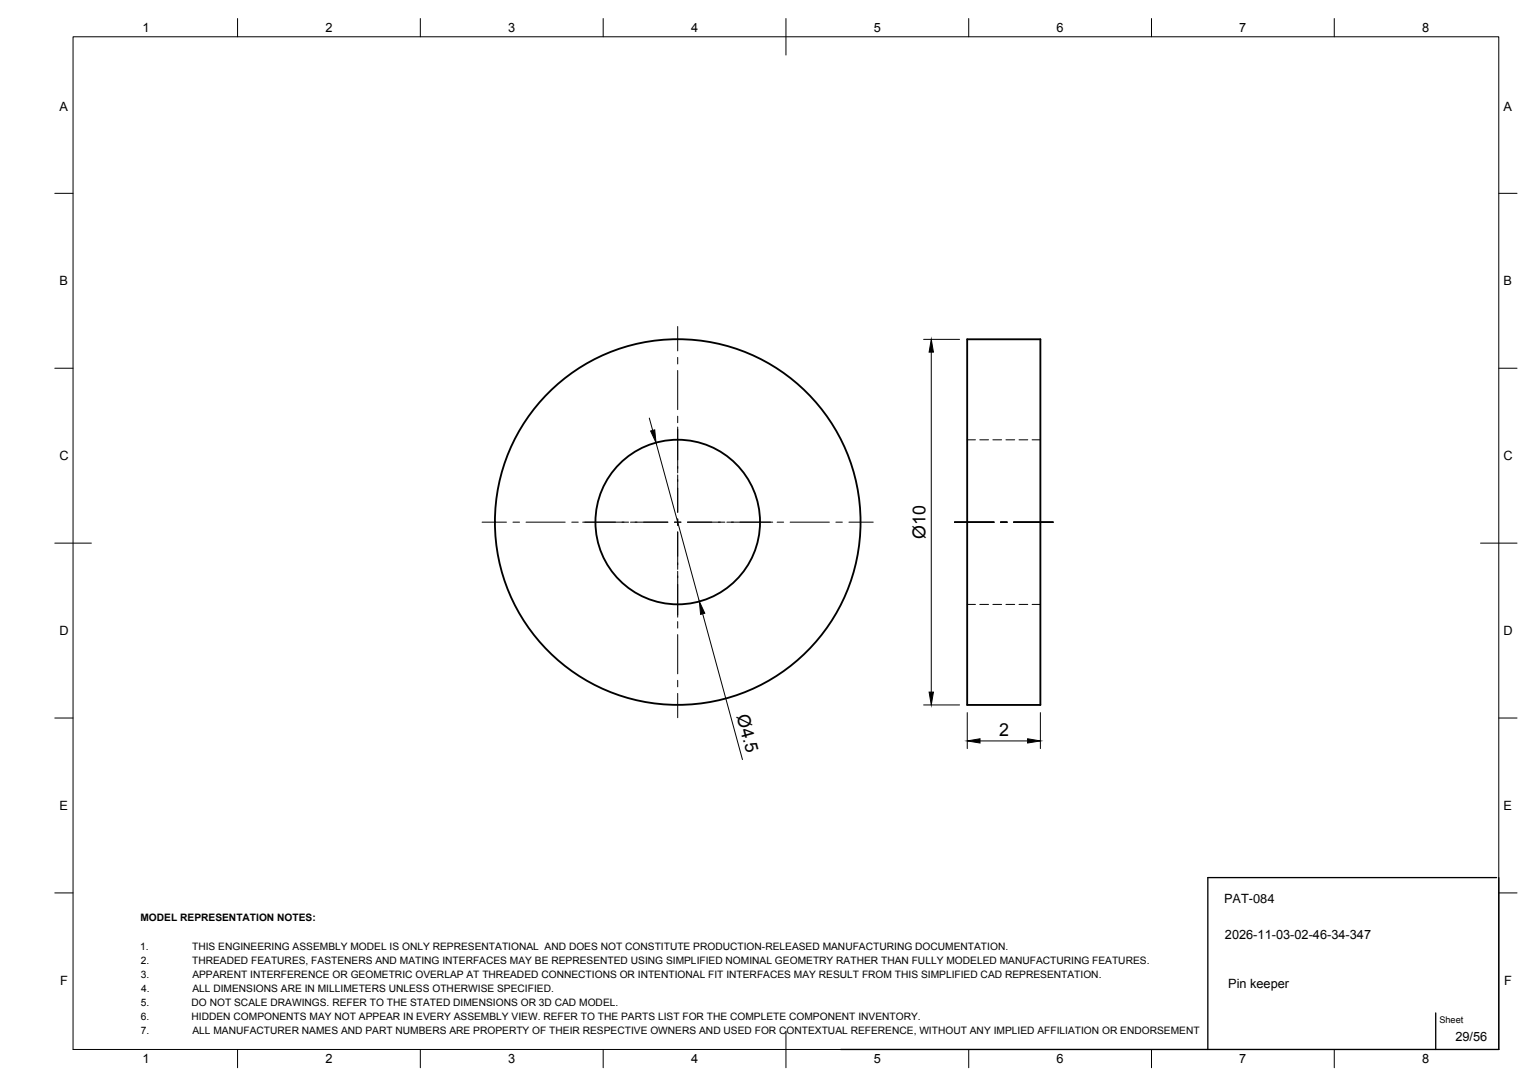
ISO-10303-21;
HEADER;
/* Generated by software containing ST-Developer
 * from STEP Tools, Inc. (www.steptools.com) 
 */

FILE_DESCRIPTION(
/* description */ ('Quick-return (Whitworth) mechanism'),
/* implementation_level */ '2;1');

FILE_NAME(
/* name */ 'Pin keeper.step',
/* time_stamp */ '2026-10-28T03:25:57-07:00',
/* author */ (''),
/* organization */ (''),
/* preprocessor_version */ 'ST-DEVELOPER v20.2',
/* originating_system */ 'Autodesk Translation Framework v15.17.0.0',
/* authorisation */ '');

FILE_SCHEMA (('AUTOMOTIVE_DESIGN { 1 0 10303 214 3 1 1 }'));
ENDSEC;

DATA;
#10=MECHANICAL_DESIGN_GEOMETRIC_PRESENTATION_REPRESENTATION('',(#518),#14878);
#422=SHAPE_REPRESENTATION_RELATIONSHIP('SRR','None',#15092,#466);
#466=ADVANCED_BREP_SHAPE_REPRESENTATION('',(#570),#14849);
#518=STYLED_ITEM('',(#15406),#570);
#570=MANIFOLD_SOLID_BREP('Body1',#7872);
#722=FACE_BOUND('',#1897,.T.);
#723=FACE_BOUND('',#1899,.T.);
#899=PLANE('',#8952);
#900=PLANE('',#8953);
#1297=FACE_OUTER_BOUND('',#1894,.T.);
#1298=FACE_OUTER_BOUND('',#1895,.T.);
#1299=FACE_OUTER_BOUND('',#1896,.T.);
#1300=FACE_OUTER_BOUND('',#1898,.T.);
#1894=EDGE_LOOP('',(#6306,#6307,#6308,#6309));
#1895=EDGE_LOOP('',(#6310,#6311,#6312,#6313));
#1896=EDGE_LOOP('',(#6314));
#1897=EDGE_LOOP('',(#6315));
#1898=EDGE_LOOP('',(#6316));
#1899=EDGE_LOOP('',(#6317));
#2379=LINE('',#13646,#2902);
#2380=LINE('',#13652,#2903);
#2902=VECTOR('',#10734,0.225);
#2903=VECTOR('',#10741,0.5);
#3498=CIRCLE('',#8947,0.225);
#3499=CIRCLE('',#8948,0.225);
#3500=CIRCLE('',#8950,0.5);
#3501=CIRCLE('',#8951,0.5);
#3990=VERTEX_POINT('',#13643);
#3991=VERTEX_POINT('',#13645);
#3992=VERTEX_POINT('',#13649);
#3993=VERTEX_POINT('',#13651);
#4810=EDGE_CURVE('',#3990,#3990,#3498,.T.);
#4811=EDGE_CURVE('',#3990,#3991,#2379,.T.);
#4812=EDGE_CURVE('',#3991,#3991,#3499,.T.);
#4813=EDGE_CURVE('',#3992,#3992,#3500,.T.);
#4814=EDGE_CURVE('',#3992,#3993,#2380,.T.);
#4815=EDGE_CURVE('',#3993,#3993,#3501,.T.);
#6306=ORIENTED_EDGE('',*,*,#4810,.F.);
#6307=ORIENTED_EDGE('',*,*,#4811,.T.);
#6308=ORIENTED_EDGE('',*,*,#4812,.T.);
#6309=ORIENTED_EDGE('',*,*,#4811,.F.);
#6310=ORIENTED_EDGE('',*,*,#4813,.F.);
#6311=ORIENTED_EDGE('',*,*,#4814,.T.);
#6312=ORIENTED_EDGE('',*,*,#4815,.T.);
#6313=ORIENTED_EDGE('',*,*,#4814,.F.);
#6314=ORIENTED_EDGE('',*,*,#4813,.T.);
#6315=ORIENTED_EDGE('',*,*,#4810,.T.);
#6316=ORIENTED_EDGE('',*,*,#4815,.F.);
#6317=ORIENTED_EDGE('',*,*,#4812,.F.);
#7321=CYLINDRICAL_SURFACE('',#8946,0.225);
#7322=CYLINDRICAL_SURFACE('',#8949,0.5);
#7628=ADVANCED_FACE('',(#1297),#7321,.F.);
#7629=ADVANCED_FACE('',(#1298),#7322,.T.);
#7630=ADVANCED_FACE('',(#1299,#722),#899,.T.);
#7631=ADVANCED_FACE('',(#1300,#723),#900,.F.);
#7872=CLOSED_SHELL('',(#7628,#7629,#7630,#7631));
#8945=AXIS2_PLACEMENT_3D('',#13641,#10728,#10729);
#8946=AXIS2_PLACEMENT_3D('',#13642,#10730,#10731);
#8947=AXIS2_PLACEMENT_3D('',#13644,#10732,#10733);
#8948=AXIS2_PLACEMENT_3D('',#13647,#10735,#10736);
#8949=AXIS2_PLACEMENT_3D('',#13648,#10737,#10738);
#8950=AXIS2_PLACEMENT_3D('',#13650,#10739,#10740);
#8951=AXIS2_PLACEMENT_3D('',#13653,#10742,#10743);
#8952=AXIS2_PLACEMENT_3D('',#13654,#10744,#10745);
#8953=AXIS2_PLACEMENT_3D('',#13655,#10746,#10747);
#10728=DIRECTION('axis',(0.,0.,1.));
#10729=DIRECTION('refdir',(1.,0.,0.));
#10730=DIRECTION('center_axis',(0.,0.,1.));
#10731=DIRECTION('ref_axis',(1.,0.,0.));
#10732=DIRECTION('center_axis',(0.,0.,-1.));
#10733=DIRECTION('ref_axis',(1.,0.,0.));
#10734=DIRECTION('',(0.,0.,-1.));
#10735=DIRECTION('center_axis',(0.,0.,-1.));
#10736=DIRECTION('ref_axis',(1.,0.,0.));
#10737=DIRECTION('center_axis',(0.,0.,1.));
#10738=DIRECTION('ref_axis',(1.,0.,0.));
#10739=DIRECTION('center_axis',(0.,0.,1.));
#10740=DIRECTION('ref_axis',(1.,0.,0.));
#10741=DIRECTION('',(0.,0.,-1.));
#10742=DIRECTION('center_axis',(0.,0.,1.));
#10743=DIRECTION('ref_axis',(1.,0.,0.));
#10744=DIRECTION('center_axis',(0.,0.,1.));
#10745=DIRECTION('ref_axis',(1.,0.,0.));
#10746=DIRECTION('center_axis',(0.,0.,1.));
#10747=DIRECTION('ref_axis',(1.,0.,0.));
#13641=CARTESIAN_POINT('',(0.,0.,0.));
#13642=CARTESIAN_POINT('Origin',(0.,9.,8.));
#13643=CARTESIAN_POINT('',(-0.225,9.,8.2));
#13644=CARTESIAN_POINT('Origin',(0.,9.,8.2));
#13645=CARTESIAN_POINT('',(-0.225,9.,8.));
#13646=CARTESIAN_POINT('',(-0.225,9.,8.));
#13647=CARTESIAN_POINT('Origin',(0.,9.,8.));
#13648=CARTESIAN_POINT('Origin',(0.,9.,8.));
#13649=CARTESIAN_POINT('',(-0.5,9.,8.2));
#13650=CARTESIAN_POINT('Origin',(0.,9.,8.2));
#13651=CARTESIAN_POINT('',(-0.5,9.,8.));
#13652=CARTESIAN_POINT('',(-0.5,9.,8.));
#13653=CARTESIAN_POINT('Origin',(0.,9.,8.));
#13654=CARTESIAN_POINT('Origin',(0.,9.,8.2));
#13655=CARTESIAN_POINT('Origin',(0.,9.,8.));
#14795=UNCERTAINTY_MEASURE_WITH_UNIT(LENGTH_MEASURE(0.001),#14879,
'DISTANCE_ACCURACY_VALUE',
'Maximum model space distance between geometric entities at asserted c
onnectivities');
#14824=UNCERTAINTY_MEASURE_WITH_UNIT(LENGTH_MEASURE(0.001),#14879,
'DISTANCE_ACCURACY_VALUE',
'Maximum model space distance between geometric entities at asserted c
onnectivities');
#14849=(
GEOMETRIC_REPRESENTATION_CONTEXT(3)
GLOBAL_UNCERTAINTY_ASSIGNED_CONTEXT((#14795))
GLOBAL_UNIT_ASSIGNED_CONTEXT((#14879,#14881,#14882))
REPRESENTATION_CONTEXT('','3D')
);
#14878=(
GEOMETRIC_REPRESENTATION_CONTEXT(3)
GLOBAL_UNCERTAINTY_ASSIGNED_CONTEXT((#14824))
GLOBAL_UNIT_ASSIGNED_CONTEXT((#14879,#14881,#14882))
REPRESENTATION_CONTEXT('','3D')
);
#14879=(
LENGTH_UNIT()
NAMED_UNIT(*)
SI_UNIT(.CENTI.,.METRE.)
);
#14881=(
NAMED_UNIT(*)
PLANE_ANGLE_UNIT()
SI_UNIT($,.RADIAN.)
);
#14882=(
NAMED_UNIT(*)
SI_UNIT($,.STERADIAN.)
SOLID_ANGLE_UNIT()
);
#14907=SHAPE_DEFINITION_REPRESENTATION(#14965,#15092);
#14965=PRODUCT_DEFINITION_SHAPE('',$,#15146);
#15092=SHAPE_REPRESENTATION('',(#8945),#14849);
#15121=PRODUCT_DEFINITION_CONTEXT('part definition',#15282,'design');
#15146=PRODUCT_DEFINITION('Pin keeper','Pin keeper',#15199,#15121);
#15199=PRODUCT_DEFINITION_FORMATION('',$,#15308);
#15282=APPLICATION_CONTEXT(
'Core Data for Automotive Mechanical Design Process');
#15283=PRODUCT_CONTEXT('part definition',#15282,'mechanical');
#15308=PRODUCT('Pin keeper','Pin keeper','Pin keeper',(#15283));
#15400=COLOUR_RGB('Grey',0.48,0.52,0.57);
#15401=FILL_AREA_STYLE_COLOUR('',#15400);
#15402=FILL_AREA_STYLE('',(#15401));
#15403=SURFACE_STYLE_FILL_AREA(#15402);
#15404=SURFACE_SIDE_STYLE('',(#15403));
#15405=SURFACE_STYLE_USAGE(.BOTH.,#15404);
#15406=PRESENTATION_STYLE_ASSIGNMENT((#15405));
ENDSEC;
END-ISO-10303-21;
